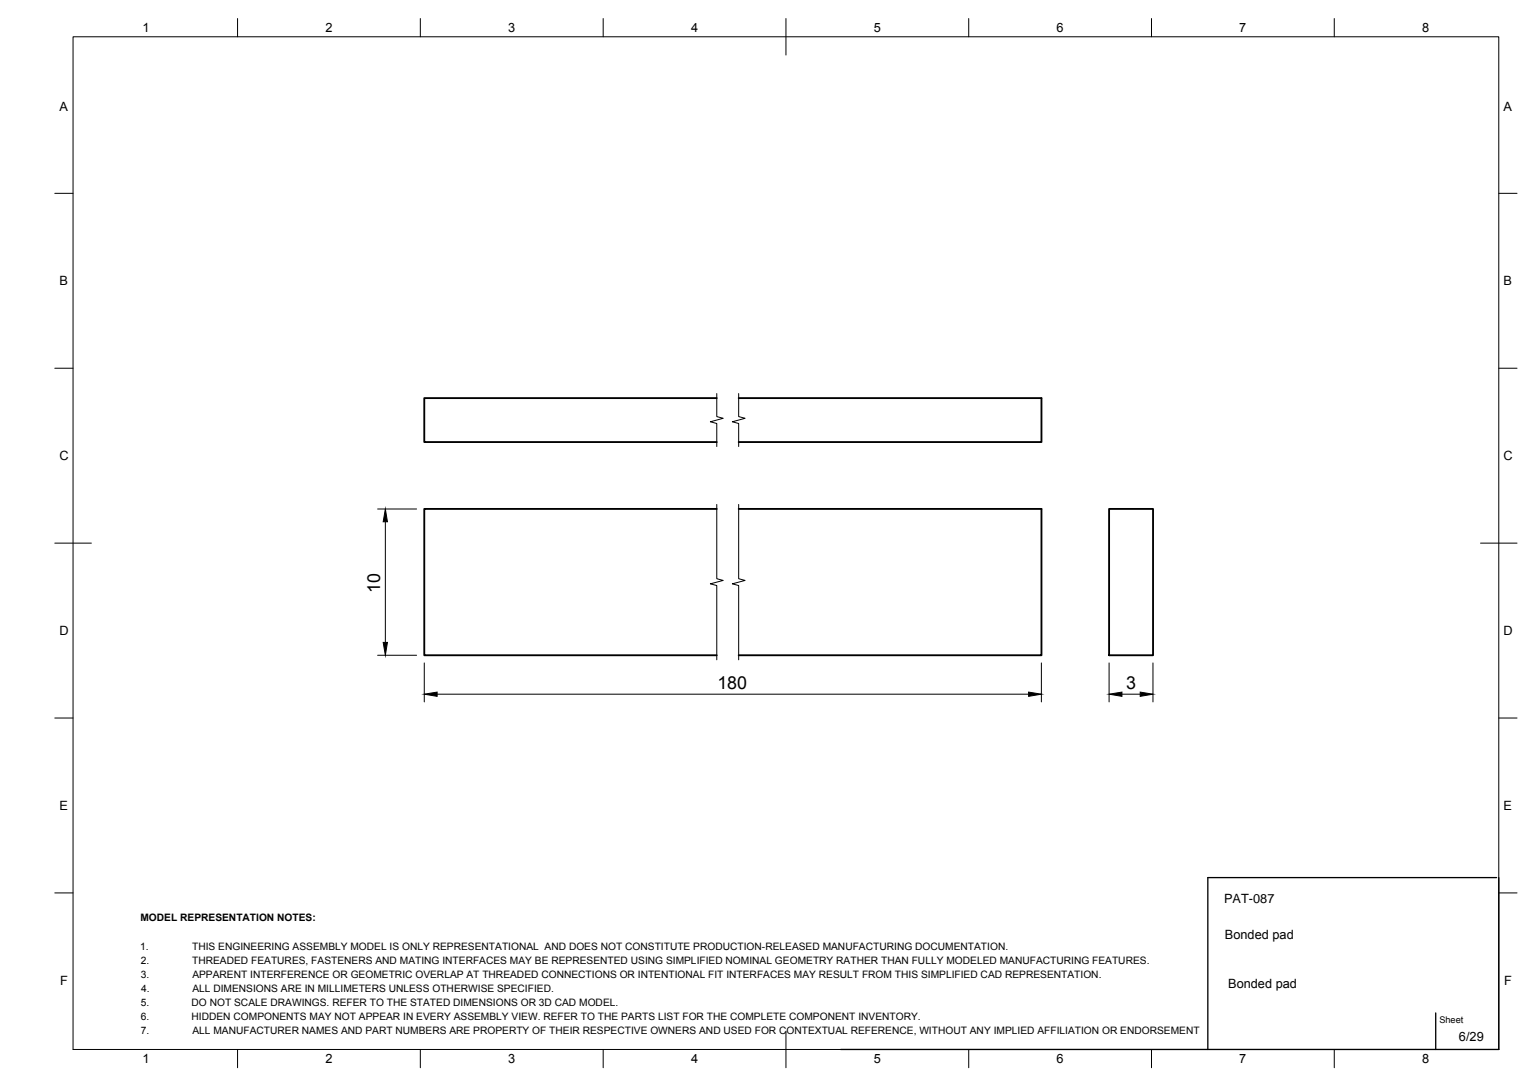
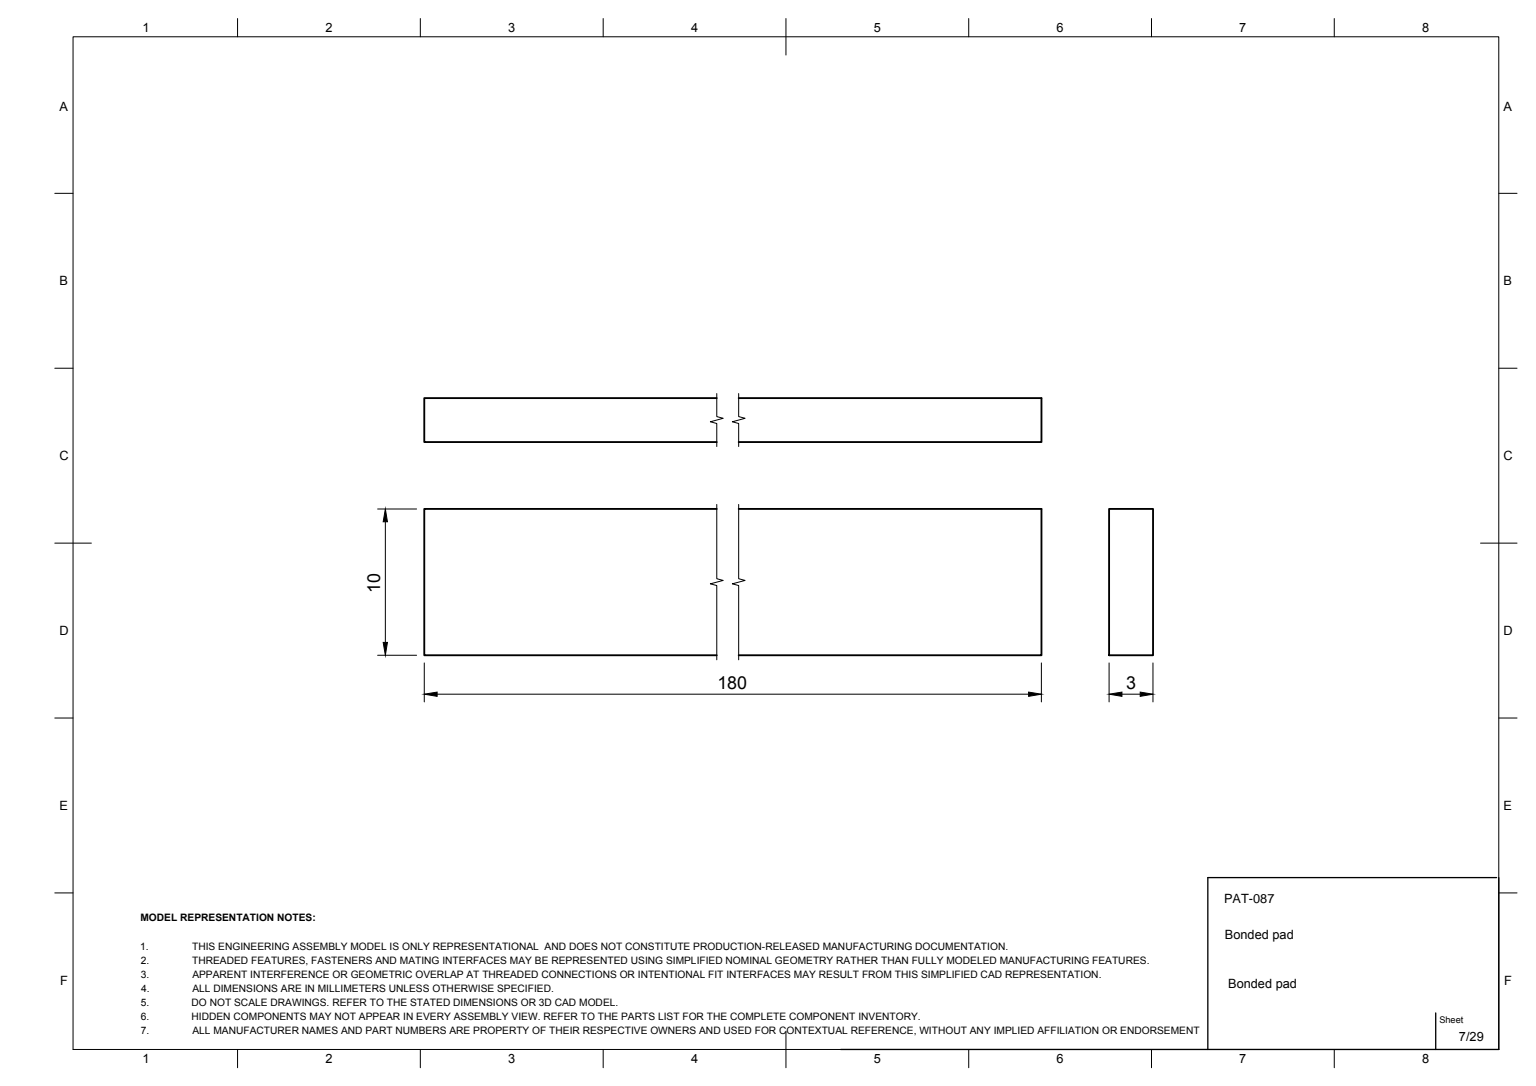
ISO-10303-21;
HEADER;
/* Generated by software containing ST-Developer
 * from STEP Tools, Inc. (www.steptools.com) 
 */

FILE_DESCRIPTION(
/* description */ ('Rigid flange shaft coupling assembly'),
/* implementation_level */ '2;1');

FILE_NAME(
/* name */ 'Bonded pad.step',
/* time_stamp */ '2026-10-27T10:47:16-07:00',
/* author */ (''),
/* organization */ (''),
/* preprocessor_version */ 'ST-DEVELOPER v20.2',
/* originating_system */ 'Autodesk Translation Framework v15.17.0.0',
/* authorisation */ '');

FILE_SCHEMA (('AUTOMOTIVE_DESIGN { 1 0 10303 214 3 1 1 }'));
ENDSEC;

DATA;
#10=MECHANICAL_DESIGN_GEOMETRIC_PRESENTATION_REPRESENTATION('',(#399),#9141);
#343=SHAPE_REPRESENTATION_RELATIONSHIP('SRR','None',#9277,#371);
#371=ADVANCED_BREP_SHAPE_REPRESENTATION('',(#428),#9112);
#399=STYLED_ITEM('',(#9514),#428);
#428=MANIFOLD_SOLID_BREP('Body1',#4753);
#576=PLANE('',#5115);
#577=PLANE('',#5116);
#578=PLANE('',#5117);
#579=PLANE('',#5118);
#580=PLANE('',#5119);
#581=PLANE('',#5120);
#754=FACE_OUTER_BOUND('',#1034,.T.);
#755=FACE_OUTER_BOUND('',#1035,.T.);
#756=FACE_OUTER_BOUND('',#1036,.T.);
#757=FACE_OUTER_BOUND('',#1037,.T.);
#758=FACE_OUTER_BOUND('',#1038,.T.);
#759=FACE_OUTER_BOUND('',#1039,.T.);
#1034=EDGE_LOOP('',(#3291,#3292,#3293,#3294));
#1035=EDGE_LOOP('',(#3295,#3296,#3297,#3298));
#1036=EDGE_LOOP('',(#3299,#3300,#3301,#3302));
#1037=EDGE_LOOP('',(#3303,#3304,#3305,#3306));
#1038=EDGE_LOOP('',(#3307,#3308,#3309,#3310));
#1039=EDGE_LOOP('',(#3311,#3312,#3313,#3314));
#1421=LINE('',#7142,#1766);
#1422=LINE('',#7144,#1767);
#1423=LINE('',#7146,#1768);
#1424=LINE('',#7147,#1769);
#1425=LINE('',#7150,#1770);
#1426=LINE('',#7152,#1771);
#1427=LINE('',#7153,#1772);
#1428=LINE('',#7156,#1773);
#1429=LINE('',#7158,#1774);
#1430=LINE('',#7159,#1775);
#1431=LINE('',#7161,#1776);
#1432=LINE('',#7162,#1777);
#1766=VECTOR('',#5704,1.);
#1767=VECTOR('',#5705,1.);
#1768=VECTOR('',#5706,1.);
#1769=VECTOR('',#5707,1.);
#1770=VECTOR('',#5710,1.);
#1771=VECTOR('',#5711,1.);
#1772=VECTOR('',#5712,1.);
#1773=VECTOR('',#5715,1.);
#1774=VECTOR('',#5716,1.);
#1775=VECTOR('',#5717,1.);
#1776=VECTOR('',#5720,1.);
#1777=VECTOR('',#5721,1.);
#2292=VERTEX_POINT('',#7140);
#2293=VERTEX_POINT('',#7141);
#2294=VERTEX_POINT('',#7143);
#2295=VERTEX_POINT('',#7145);
#2296=VERTEX_POINT('',#7149);
#2297=VERTEX_POINT('',#7151);
#2298=VERTEX_POINT('',#7155);
#2299=VERTEX_POINT('',#7157);
#2689=EDGE_CURVE('',#2292,#2293,#1421,.T.);
#2690=EDGE_CURVE('',#2293,#2294,#1422,.T.);
#2691=EDGE_CURVE('',#2295,#2294,#1423,.T.);
#2692=EDGE_CURVE('',#2292,#2295,#1424,.T.);
#2693=EDGE_CURVE('',#2296,#2292,#1425,.T.);
#2694=EDGE_CURVE('',#2297,#2295,#1426,.T.);
#2695=EDGE_CURVE('',#2296,#2297,#1427,.T.);
#2696=EDGE_CURVE('',#2298,#2296,#1428,.T.);
#2697=EDGE_CURVE('',#2299,#2297,#1429,.T.);
#2698=EDGE_CURVE('',#2298,#2299,#1430,.T.);
#2699=EDGE_CURVE('',#2293,#2298,#1431,.T.);
#2700=EDGE_CURVE('',#2294,#2299,#1432,.T.);
#3291=ORIENTED_EDGE('',*,*,#2689,.T.);
#3292=ORIENTED_EDGE('',*,*,#2690,.T.);
#3293=ORIENTED_EDGE('',*,*,#2691,.F.);
#3294=ORIENTED_EDGE('',*,*,#2692,.F.);
#3295=ORIENTED_EDGE('',*,*,#2693,.T.);
#3296=ORIENTED_EDGE('',*,*,#2692,.T.);
#3297=ORIENTED_EDGE('',*,*,#2694,.F.);
#3298=ORIENTED_EDGE('',*,*,#2695,.F.);
#3299=ORIENTED_EDGE('',*,*,#2696,.T.);
#3300=ORIENTED_EDGE('',*,*,#2695,.T.);
#3301=ORIENTED_EDGE('',*,*,#2697,.F.);
#3302=ORIENTED_EDGE('',*,*,#2698,.F.);
#3303=ORIENTED_EDGE('',*,*,#2699,.T.);
#3304=ORIENTED_EDGE('',*,*,#2698,.T.);
#3305=ORIENTED_EDGE('',*,*,#2700,.F.);
#3306=ORIENTED_EDGE('',*,*,#2690,.F.);
#3307=ORIENTED_EDGE('',*,*,#2700,.T.);
#3308=ORIENTED_EDGE('',*,*,#2697,.T.);
#3309=ORIENTED_EDGE('',*,*,#2694,.T.);
#3310=ORIENTED_EDGE('',*,*,#2691,.T.);
#3311=ORIENTED_EDGE('',*,*,#2699,.F.);
#3312=ORIENTED_EDGE('',*,*,#2689,.F.);
#3313=ORIENTED_EDGE('',*,*,#2693,.F.);
#3314=ORIENTED_EDGE('',*,*,#2696,.F.);
#4490=ADVANCED_FACE('',(#754),#576,.T.);
#4491=ADVANCED_FACE('',(#755),#577,.T.);
#4492=ADVANCED_FACE('',(#756),#578,.T.);
#4493=ADVANCED_FACE('',(#757),#579,.T.);
#4494=ADVANCED_FACE('',(#758),#580,.T.);
#4495=ADVANCED_FACE('',(#759),#581,.F.);
#4753=CLOSED_SHELL('',(#4490,#4491,#4492,#4493,#4494,#4495));
#5114=AXIS2_PLACEMENT_3D('',#7138,#5700,#5701);
#5115=AXIS2_PLACEMENT_3D('',#7139,#5702,#5703);
#5116=AXIS2_PLACEMENT_3D('',#7148,#5708,#5709);
#5117=AXIS2_PLACEMENT_3D('',#7154,#5713,#5714);
#5118=AXIS2_PLACEMENT_3D('',#7160,#5718,#5719);
#5119=AXIS2_PLACEMENT_3D('',#7163,#5722,#5723);
#5120=AXIS2_PLACEMENT_3D('',#7164,#5724,#5725);
#5700=DIRECTION('axis',(0.,0.,1.));
#5701=DIRECTION('refdir',(1.,0.,0.));
#5702=DIRECTION('center_axis',(0.,1.,0.));
#5703=DIRECTION('ref_axis',(-1.,0.,0.));
#5704=DIRECTION('',(-1.,0.,0.));
#5705=DIRECTION('',(0.,0.,1.));
#5706=DIRECTION('',(-1.,0.,0.));
#5707=DIRECTION('',(0.,0.,1.));
#5708=DIRECTION('center_axis',(1.,0.,0.));
#5709=DIRECTION('ref_axis',(0.,1.,0.));
#5710=DIRECTION('',(0.,1.,0.));
#5711=DIRECTION('',(0.,1.,0.));
#5712=DIRECTION('',(0.,0.,1.));
#5713=DIRECTION('center_axis',(0.,-1.,0.));
#5714=DIRECTION('ref_axis',(1.,0.,0.));
#5715=DIRECTION('',(1.,0.,0.));
#5716=DIRECTION('',(1.,0.,0.));
#5717=DIRECTION('',(0.,0.,1.));
#5718=DIRECTION('center_axis',(-1.,0.,0.));
#5719=DIRECTION('ref_axis',(0.,-1.,0.));
#5720=DIRECTION('',(0.,-1.,0.));
#5721=DIRECTION('',(0.,-1.,0.));
#5722=DIRECTION('center_axis',(0.,0.,1.));
#5723=DIRECTION('ref_axis',(1.,0.,0.));
#5724=DIRECTION('center_axis',(0.,0.,1.));
#5725=DIRECTION('ref_axis',(1.,0.,0.));
#7138=CARTESIAN_POINT('',(0.,0.,0.));
#7139=CARTESIAN_POINT('Origin',(9.,-3.,-0.3));
#7140=CARTESIAN_POINT('',(9.,-3.,-0.3));
#7141=CARTESIAN_POINT('',(-9.,-3.,-0.3));
#7142=CARTESIAN_POINT('',(9.,-3.,-0.3));
#7143=CARTESIAN_POINT('',(-9.,-3.,0.));
#7144=CARTESIAN_POINT('',(-9.,-3.,-0.3));
#7145=CARTESIAN_POINT('',(9.,-3.,0.));
#7146=CARTESIAN_POINT('',(9.,-3.,0.));
#7147=CARTESIAN_POINT('',(9.,-3.,-0.3));
#7148=CARTESIAN_POINT('Origin',(9.,-4.,-0.3));
#7149=CARTESIAN_POINT('',(9.,-4.,-0.3));
#7150=CARTESIAN_POINT('',(9.,-4.,-0.3));
#7151=CARTESIAN_POINT('',(9.,-4.,0.));
#7152=CARTESIAN_POINT('',(9.,-4.,0.));
#7153=CARTESIAN_POINT('',(9.,-4.,-0.3));
#7154=CARTESIAN_POINT('Origin',(-9.,-4.,-0.3));
#7155=CARTESIAN_POINT('',(-9.,-4.,-0.3));
#7156=CARTESIAN_POINT('',(-9.,-4.,-0.3));
#7157=CARTESIAN_POINT('',(-9.,-4.,0.));
#7158=CARTESIAN_POINT('',(-9.,-4.,0.));
#7159=CARTESIAN_POINT('',(-9.,-4.,-0.3));
#7160=CARTESIAN_POINT('Origin',(-9.,-3.,-0.3));
#7161=CARTESIAN_POINT('',(-9.,-3.,-0.3));
#7162=CARTESIAN_POINT('',(-9.,-3.,0.));
#7163=CARTESIAN_POINT('Origin',(0.,-3.5,0.));
#7164=CARTESIAN_POINT('Origin',(0.,-3.5,-0.3));
#9079=UNCERTAINTY_MEASURE_WITH_UNIT(LENGTH_MEASURE(0.001),#9142,
'DISTANCE_ACCURACY_VALUE',
'Maximum model space distance between geometric entities at asserted c
onnectivities');
#9108=UNCERTAINTY_MEASURE_WITH_UNIT(LENGTH_MEASURE(0.001),#9142,
'DISTANCE_ACCURACY_VALUE',
'Maximum model space distance between geometric entities at asserted c
onnectivities');
#9112=(
GEOMETRIC_REPRESENTATION_CONTEXT(3)
GLOBAL_UNCERTAINTY_ASSIGNED_CONTEXT((#9079))
GLOBAL_UNIT_ASSIGNED_CONTEXT((#9142,#9144,#9145))
REPRESENTATION_CONTEXT('','3D')
);
#9141=(
GEOMETRIC_REPRESENTATION_CONTEXT(3)
GLOBAL_UNCERTAINTY_ASSIGNED_CONTEXT((#9108))
GLOBAL_UNIT_ASSIGNED_CONTEXT((#9142,#9144,#9145))
REPRESENTATION_CONTEXT('','3D')
);
#9142=(
LENGTH_UNIT()
NAMED_UNIT(*)
SI_UNIT(.CENTI.,.METRE.)
);
#9144=(
NAMED_UNIT(*)
PLANE_ANGLE_UNIT()
SI_UNIT($,.RADIAN.)
);
#9145=(
NAMED_UNIT(*)
SI_UNIT($,.STERADIAN.)
SOLID_ANGLE_UNIT()
);
#9149=SHAPE_DEFINITION_REPRESENTATION(#9181,#9277);
#9181=PRODUCT_DEFINITION_SHAPE('',$,#9310);
#9277=SHAPE_REPRESENTATION('',(#5114),#9112);
#9306=PRODUCT_DEFINITION_CONTEXT('part definition',#9404,'design');
#9310=PRODUCT_DEFINITION('Bonded pad','Bonded pad',#9342,#9306);
#9342=PRODUCT_DEFINITION_FORMATION('',$,#9409);
#9404=APPLICATION_CONTEXT(
'Core Data for Automotive Mechanical Design Process');
#9405=PRODUCT_CONTEXT('part definition',#9404,'mechanical');
#9409=PRODUCT('Bonded pad','Bonded pad','Bonded pad',(#9405));
#9508=COLOUR_RGB('Off White',0.89,0.88,0.83);
#9509=FILL_AREA_STYLE_COLOUR('',#9508);
#9510=FILL_AREA_STYLE('',(#9509));
#9511=SURFACE_STYLE_FILL_AREA(#9510);
#9512=SURFACE_SIDE_STYLE('',(#9511));
#9513=SURFACE_STYLE_USAGE(.BOTH.,#9512);
#9514=PRESENTATION_STYLE_ASSIGNMENT((#9513));
ENDSEC;
END-ISO-10303-21;
